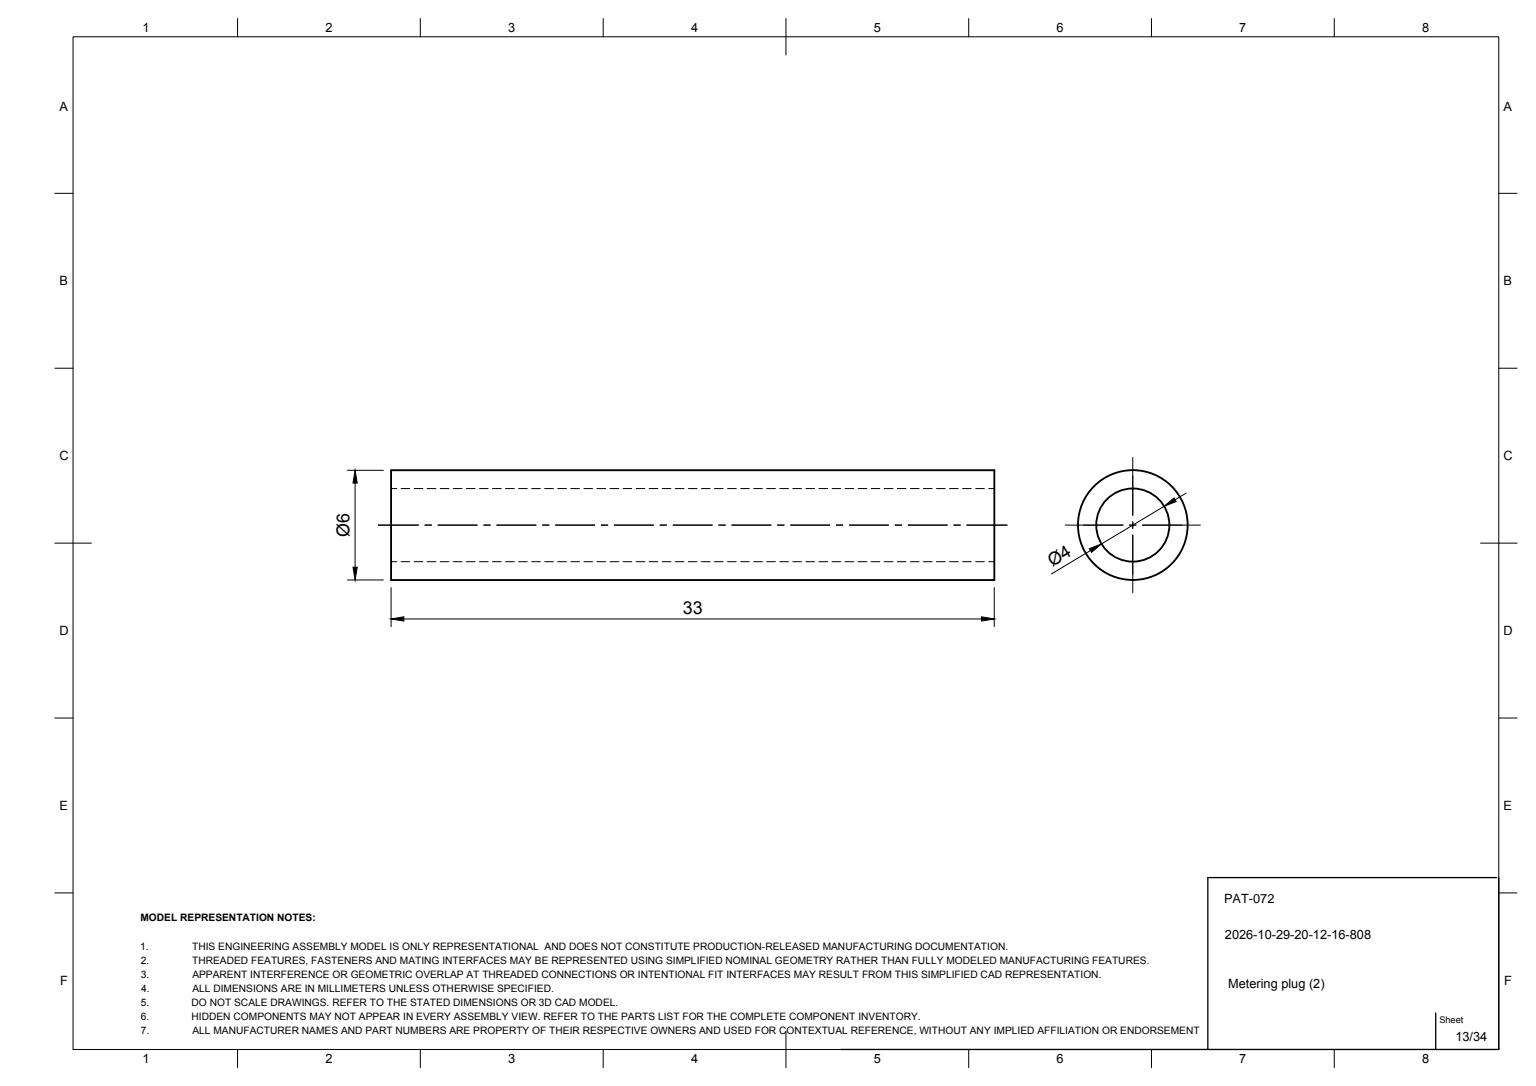
ISO-10303-21;
HEADER;
/* Generated by software containing ST-Developer
 * from STEP Tools, Inc. (www.steptools.com) 
 */

FILE_DESCRIPTION(
/* description */ ('PAT-072'),
/* implementation_level */ '2;1');

FILE_NAME(
/* name */ 'Metering plug (2).step',
/* time_stamp */ '2026-10-29T20:11:56-07:00',
/* author */ (''),
/* organization */ (''),
/* preprocessor_version */ 'ST-DEVELOPER v20.2',
/* originating_system */ 'Autodesk Translation Framework v15.17.0.0',
/* authorisation */ '');

FILE_SCHEMA (('AUTOMOTIVE_DESIGN { 1 0 10303 214 3 1 1 }'));
ENDSEC;

DATA;
#10=MECHANICAL_DESIGN_GEOMETRIC_PRESENTATION_REPRESENTATION('',(#343),#11432);
#271=SHAPE_REPRESENTATION_RELATIONSHIP('SRR','None',#11575,#307);
#307=ADVANCED_BREP_SHAPE_REPRESENTATION('',(#379),#11406);
#343=STYLED_ITEM('',(#11812),#379);
#379=MANIFOLD_SOLID_BREP('Body1',#6078);
#474=FACE_BOUND('',#1372,.T.);
#475=FACE_BOUND('',#1376,.T.);
#639=PLANE('',#6766);
#640=PLANE('',#6771);
#641=PLANE('',#6772);
#642=PLANE('',#6778);
#927=FACE_OUTER_BOUND('',#1371,.T.);
#928=FACE_OUTER_BOUND('',#1373,.T.);
#929=FACE_OUTER_BOUND('',#1374,.T.);
#930=FACE_OUTER_BOUND('',#1375,.T.);
#931=FACE_OUTER_BOUND('',#1377,.T.);
#932=FACE_OUTER_BOUND('',#1378,.T.);
#933=FACE_OUTER_BOUND('',#1379,.T.);
#1371=EDGE_LOOP('',(#4594));
#1372=EDGE_LOOP('',(#4595));
#1373=EDGE_LOOP('',(#4596,#4597,#4598,#4599));
#1374=EDGE_LOOP('',(#4600));
#1375=EDGE_LOOP('',(#4601));
#1376=EDGE_LOOP('',(#4602));
#1377=EDGE_LOOP('',(#4603,#4604,#4605,#4606));
#1378=EDGE_LOOP('',(#4607,#4608,#4609,#4610));
#1379=EDGE_LOOP('',(#4611));
#1826=LINE('',#10118,#2245);
#1827=LINE('',#10126,#2246);
#1828=LINE('',#10129,#2247);
#2245=VECTOR('',#7915,0.6);
#2246=VECTOR('',#7926,0.3);
#2247=VECTOR('',#7929,0.1);
#2659=CIRCLE('',#6767,0.6);
#2660=CIRCLE('',#6768,0.3);
#2661=CIRCLE('',#6770,0.6);
#2662=CIRCLE('',#6773,0.3);
#2663=CIRCLE('',#6774,0.1);
#2664=CIRCLE('',#6777,0.1);
#3008=VERTEX_POINT('',#10111);
#3009=VERTEX_POINT('',#10113);
#3010=VERTEX_POINT('',#10116);
#3011=VERTEX_POINT('',#10121);
#3012=VERTEX_POINT('',#10123);
#3013=VERTEX_POINT('',#10128);
#3586=EDGE_CURVE('',#3008,#3008,#2659,.T.);
#3587=EDGE_CURVE('',#3009,#3009,#2660,.T.);
#3588=EDGE_CURVE('',#3010,#3010,#2661,.T.);
#3589=EDGE_CURVE('',#3010,#3008,#1826,.T.);
#3590=EDGE_CURVE('',#3011,#3011,#2662,.T.);
#3591=EDGE_CURVE('',#3012,#3012,#2663,.T.);
#3592=EDGE_CURVE('',#3009,#3011,#1827,.T.);
#3593=EDGE_CURVE('',#3012,#3013,#1828,.T.);
#3594=EDGE_CURVE('',#3013,#3013,#2664,.T.);
#4594=ORIENTED_EDGE('',*,*,#3586,.F.);
#4595=ORIENTED_EDGE('',*,*,#3587,.T.);
#4596=ORIENTED_EDGE('',*,*,#3588,.F.);
#4597=ORIENTED_EDGE('',*,*,#3589,.T.);
#4598=ORIENTED_EDGE('',*,*,#3586,.T.);
#4599=ORIENTED_EDGE('',*,*,#3589,.F.);
#4600=ORIENTED_EDGE('',*,*,#3588,.T.);
#4601=ORIENTED_EDGE('',*,*,#3590,.F.);
#4602=ORIENTED_EDGE('',*,*,#3591,.T.);
#4603=ORIENTED_EDGE('',*,*,#3587,.F.);
#4604=ORIENTED_EDGE('',*,*,#3592,.T.);
#4605=ORIENTED_EDGE('',*,*,#3590,.T.);
#4606=ORIENTED_EDGE('',*,*,#3592,.F.);
#4607=ORIENTED_EDGE('',*,*,#3591,.F.);
#4608=ORIENTED_EDGE('',*,*,#3593,.T.);
#4609=ORIENTED_EDGE('',*,*,#3594,.T.);
#4610=ORIENTED_EDGE('',*,*,#3593,.F.);
#4611=ORIENTED_EDGE('',*,*,#3594,.F.);
#5620=CYLINDRICAL_SURFACE('',#6769,0.6);
#5621=CYLINDRICAL_SURFACE('',#6775,0.3);
#5622=CYLINDRICAL_SURFACE('',#6776,0.1);
#5826=ADVANCED_FACE('',(#927,#474),#639,.F.);
#5827=ADVANCED_FACE('',(#928),#5620,.T.);
#5828=ADVANCED_FACE('',(#929),#640,.T.);
#5829=ADVANCED_FACE('',(#930,#475),#641,.F.);
#5830=ADVANCED_FACE('',(#931),#5621,.T.);
#5831=ADVANCED_FACE('',(#932),#5622,.T.);
#5832=ADVANCED_FACE('',(#933),#642,.F.);
#6078=CLOSED_SHELL('',(#5826,#5827,#5828,#5829,#5830,#5831,#5832));
#6765=AXIS2_PLACEMENT_3D('',#10109,#7903,#7904);
#6766=AXIS2_PLACEMENT_3D('',#10110,#7905,#7906);
#6767=AXIS2_PLACEMENT_3D('',#10112,#7907,#7908);
#6768=AXIS2_PLACEMENT_3D('',#10114,#7909,#7910);
#6769=AXIS2_PLACEMENT_3D('',#10115,#7911,#7912);
#6770=AXIS2_PLACEMENT_3D('',#10117,#7913,#7914);
#6771=AXIS2_PLACEMENT_3D('',#10119,#7916,#7917);
#6772=AXIS2_PLACEMENT_3D('',#10120,#7918,#7919);
#6773=AXIS2_PLACEMENT_3D('',#10122,#7920,#7921);
#6774=AXIS2_PLACEMENT_3D('',#10124,#7922,#7923);
#6775=AXIS2_PLACEMENT_3D('',#10125,#7924,#7925);
#6776=AXIS2_PLACEMENT_3D('',#10127,#7927,#7928);
#6777=AXIS2_PLACEMENT_3D('',#10130,#7930,#7931);
#6778=AXIS2_PLACEMENT_3D('',#10131,#7932,#7933);
#7903=DIRECTION('axis',(0.,0.,1.));
#7904=DIRECTION('refdir',(1.,0.,0.));
#7905=DIRECTION('center_axis',(0.,0.,1.));
#7906=DIRECTION('ref_axis',(1.,0.,0.));
#7907=DIRECTION('center_axis',(0.,0.,1.));
#7908=DIRECTION('ref_axis',(1.,0.,0.));
#7909=DIRECTION('center_axis',(0.,0.,1.));
#7910=DIRECTION('ref_axis',(1.,0.,0.));
#7911=DIRECTION('center_axis',(0.,0.,1.));
#7912=DIRECTION('ref_axis',(1.,0.,0.));
#7913=DIRECTION('center_axis',(0.,0.,1.));
#7914=DIRECTION('ref_axis',(1.,0.,0.));
#7915=DIRECTION('',(0.,0.,-1.));
#7916=DIRECTION('center_axis',(0.,0.,1.));
#7917=DIRECTION('ref_axis',(1.,0.,0.));
#7918=DIRECTION('center_axis',(0.,0.,1.));
#7919=DIRECTION('ref_axis',(1.,0.,0.));
#7920=DIRECTION('center_axis',(0.,0.,1.));
#7921=DIRECTION('ref_axis',(1.,0.,0.));
#7922=DIRECTION('center_axis',(0.,0.,1.));
#7923=DIRECTION('ref_axis',(1.,0.,0.));
#7924=DIRECTION('center_axis',(0.,0.,1.));
#7925=DIRECTION('ref_axis',(1.,0.,0.));
#7926=DIRECTION('',(0.,0.,-1.));
#7927=DIRECTION('center_axis',(0.,0.,1.));
#7928=DIRECTION('ref_axis',(1.,0.,0.));
#7929=DIRECTION('',(0.,0.,-1.));
#7930=DIRECTION('center_axis',(0.,0.,1.));
#7931=DIRECTION('ref_axis',(1.,0.,0.));
#7932=DIRECTION('center_axis',(0.,0.,1.));
#7933=DIRECTION('ref_axis',(1.,0.,0.));
#10109=CARTESIAN_POINT('',(0.,0.,0.));
#10110=CARTESIAN_POINT('Origin',(1.25,1.5,6.1));
#10111=CARTESIAN_POINT('',(0.65,1.5,6.1));
#10112=CARTESIAN_POINT('Origin',(1.25,1.5,6.1));
#10113=CARTESIAN_POINT('',(0.95,1.5,6.1));
#10114=CARTESIAN_POINT('Origin',(1.25,1.5,6.1));
#10115=CARTESIAN_POINT('Origin',(1.25,1.5,6.1));
#10116=CARTESIAN_POINT('',(0.65,1.5,6.5));
#10117=CARTESIAN_POINT('Origin',(1.25,1.5,6.5));
#10118=CARTESIAN_POINT('',(0.65,1.5,6.1));
#10119=CARTESIAN_POINT('Origin',(1.25,1.5,6.5));
#10120=CARTESIAN_POINT('Origin',(1.25,1.5,4.8));
#10121=CARTESIAN_POINT('',(0.95,1.5,4.8));
#10122=CARTESIAN_POINT('Origin',(1.25,1.5,4.8));
#10123=CARTESIAN_POINT('',(1.15,1.5,4.8));
#10124=CARTESIAN_POINT('Origin',(1.25,1.5,4.8));
#10125=CARTESIAN_POINT('Origin',(1.25,1.5,4.8));
#10126=CARTESIAN_POINT('',(0.95,1.5,4.8));
#10127=CARTESIAN_POINT('Origin',(1.25,1.5,4.1));
#10128=CARTESIAN_POINT('',(1.15,1.5,4.1));
#10129=CARTESIAN_POINT('',(1.15,1.5,4.1));
#10130=CARTESIAN_POINT('Origin',(1.25,1.5,4.1));
#10131=CARTESIAN_POINT('Origin',(1.25,1.5,4.1));
#11367=UNCERTAINTY_MEASURE_WITH_UNIT(LENGTH_MEASURE(0.001),#11433,
'DISTANCE_ACCURACY_VALUE',
'Maximum model space distance between geometric entities at asserted c
onnectivities');
#11393=UNCERTAINTY_MEASURE_WITH_UNIT(LENGTH_MEASURE(0.001),#11433,
'DISTANCE_ACCURACY_VALUE',
'Maximum model space distance between geometric entities at asserted c
onnectivities');
#11406=(
GEOMETRIC_REPRESENTATION_CONTEXT(3)
GLOBAL_UNCERTAINTY_ASSIGNED_CONTEXT((#11367))
GLOBAL_UNIT_ASSIGNED_CONTEXT((#11433,#11435,#11436))
REPRESENTATION_CONTEXT('','3D')
);
#11432=(
GEOMETRIC_REPRESENTATION_CONTEXT(3)
GLOBAL_UNCERTAINTY_ASSIGNED_CONTEXT((#11393))
GLOBAL_UNIT_ASSIGNED_CONTEXT((#11433,#11435,#11436))
REPRESENTATION_CONTEXT('','3D')
);
#11433=(
LENGTH_UNIT()
NAMED_UNIT(*)
SI_UNIT(.CENTI.,.METRE.)
);
#11435=(
NAMED_UNIT(*)
PLANE_ANGLE_UNIT()
SI_UNIT($,.RADIAN.)
);
#11436=(
NAMED_UNIT(*)
SI_UNIT($,.STERADIAN.)
SOLID_ANGLE_UNIT()
);
#11449=SHAPE_DEFINITION_REPRESENTATION(#11487,#11575);
#11487=PRODUCT_DEFINITION_SHAPE('',$,#11614);
#11575=SHAPE_REPRESENTATION('',(#6765),#11406);
#11601=PRODUCT_DEFINITION_CONTEXT('part definition',#11717,'design');
#11614=PRODUCT_DEFINITION('Metering plug (2)',
'Metering plug (2)',#11652,#11601);
#11652=PRODUCT_DEFINITION_FORMATION('',$,#11731);
#11717=APPLICATION_CONTEXT(
'Core Data for Automotive Mechanical Design Process');
#11718=PRODUCT_CONTEXT('part definition',#11717,'mechanical');
#11731=PRODUCT('Metering plug (2)','Metering plug (2)',
'Metering plug (2)',(#11718));
#11806=COLOUR_RGB('Sky Blue',0.24,0.69,0.87);
#11807=FILL_AREA_STYLE_COLOUR('',#11806);
#11808=FILL_AREA_STYLE('',(#11807));
#11809=SURFACE_STYLE_FILL_AREA(#11808);
#11810=SURFACE_SIDE_STYLE('',(#11809));
#11811=SURFACE_STYLE_USAGE(.BOTH.,#11810);
#11812=PRESENTATION_STYLE_ASSIGNMENT((#11811));
ENDSEC;
END-ISO-10303-21;
